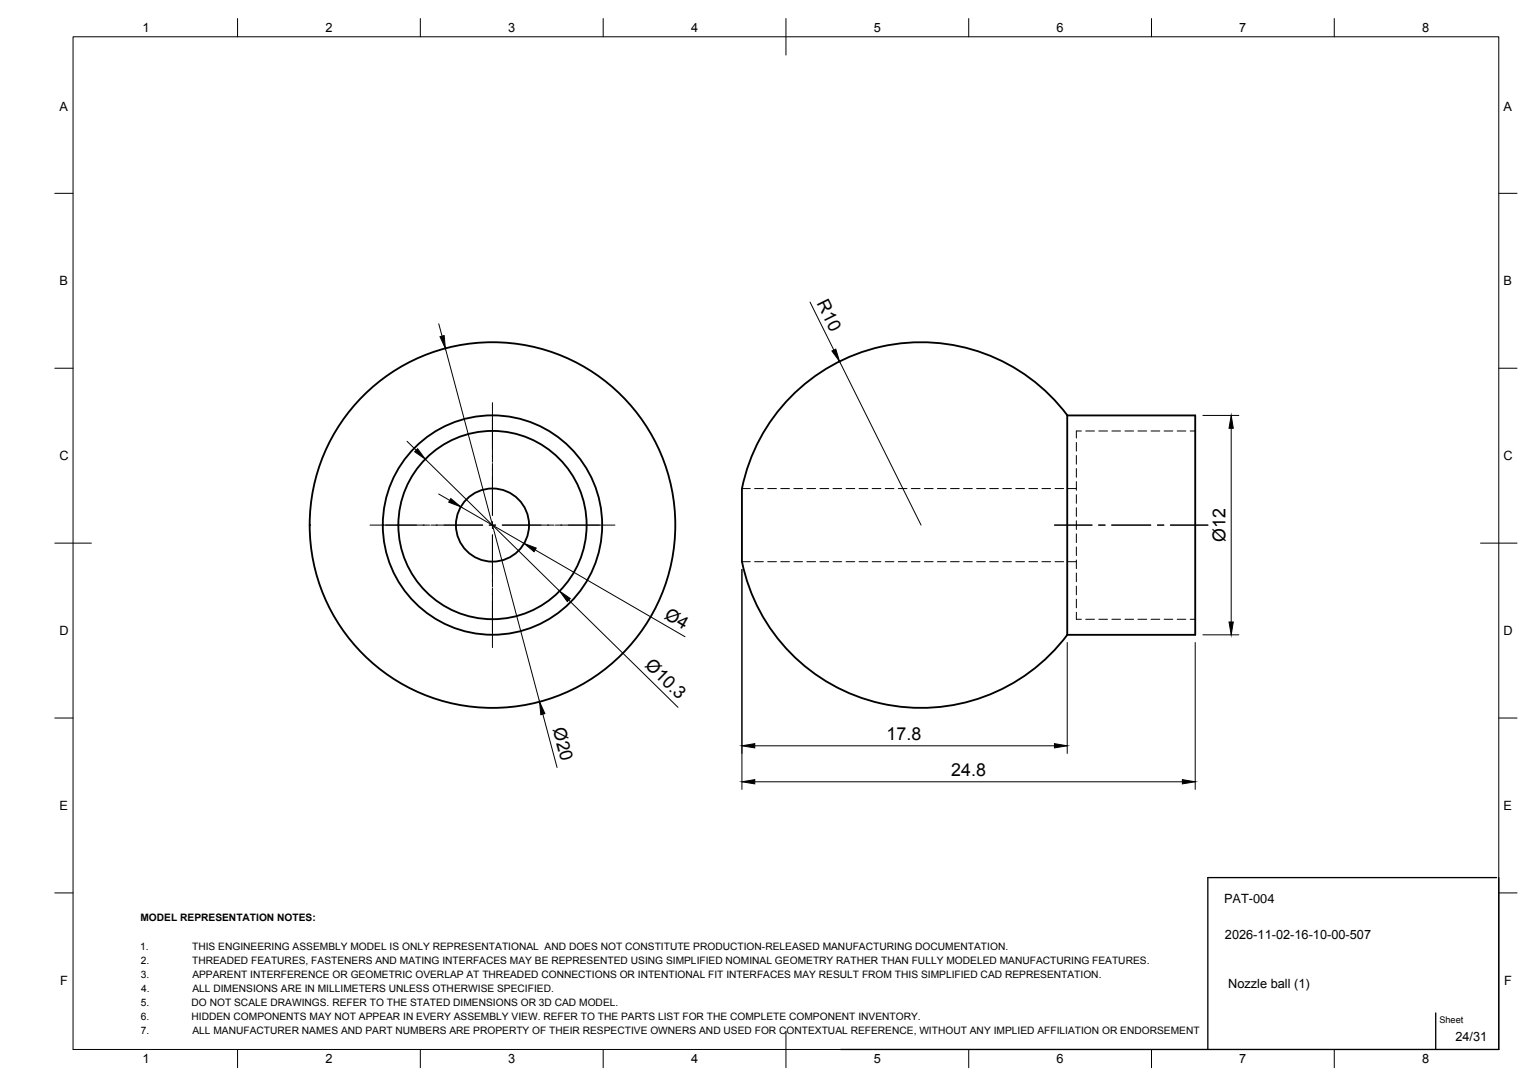
ISO-10303-21;
HEADER;
/* Generated by software containing ST-Developer
 * from STEP Tools, Inc. (www.steptools.com) 
 */

FILE_DESCRIPTION(
/* description */ ('Air blow-off nozzle station'),
/* implementation_level */ '2;1');

FILE_NAME(
/* name */ 'Nozzle ball (1).step',
/* time_stamp */ '2026-10-27T10:53:54-07:00',
/* author */ (''),
/* organization */ (''),
/* preprocessor_version */ 'ST-DEVELOPER v20.2',
/* originating_system */ 'Autodesk Translation Framework v15.17.0.0',
/* authorisation */ '');

FILE_SCHEMA (('AUTOMOTIVE_DESIGN { 1 0 10303 214 3 1 1 }'));
ENDSEC;

DATA;
#10=MECHANICAL_DESIGN_GEOMETRIC_PRESENTATION_REPRESENTATION('',(#254),#7897);
#169=SPHERICAL_SURFACE('',#4951,1.);
#204=SHAPE_REPRESENTATION_RELATIONSHIP('SRR','None',#8020,#229);
#229=ADVANCED_BREP_SHAPE_REPRESENTATION('',(#277),#7887);
#254=STYLED_ITEM('',(#8234),#277);
#277=MANIFOLD_SOLID_BREP('Body1',#4305);
#344=FACE_BOUND('',#1058,.T.);
#345=FACE_BOUND('',#1062,.T.);
#346=FACE_BOUND('',#1064,.T.);
#347=FACE_BOUND('',#1065,.T.);
#511=PLANE('',#4943);
#512=PLANE('',#4950);
#741=FACE_OUTER_BOUND('',#1056,.T.);
#742=FACE_OUTER_BOUND('',#1057,.T.);
#743=FACE_OUTER_BOUND('',#1059,.T.);
#744=FACE_OUTER_BOUND('',#1060,.T.);
#745=FACE_OUTER_BOUND('',#1061,.T.);
#746=FACE_OUTER_BOUND('',#1063,.T.);
#1056=EDGE_LOOP('',(#3775,#3776,#3777,#3778));
#1057=EDGE_LOOP('',(#3779));
#1058=EDGE_LOOP('',(#3780));
#1059=EDGE_LOOP('',(#3781,#3782,#3783,#3784));
#1060=EDGE_LOOP('',(#3785,#3786,#3787,#3788));
#1061=EDGE_LOOP('',(#3789));
#1062=EDGE_LOOP('',(#3790));
#1063=EDGE_LOOP('',(#3791,#3792));
#1064=EDGE_LOOP('',(#3793));
#1065=EDGE_LOOP('',(#3794));
#1450=LINE('',#7600,#1804);
#1451=LINE('',#7607,#1805);
#1452=LINE('',#7613,#1806);
#1804=VECTOR('',#6090,0.515);
#1805=VECTOR('',#6099,0.2);
#1806=VECTOR('',#6106,0.6);
#1957=CIRCLE('',#4941,0.515);
#1958=CIRCLE('',#4942,0.515);
#1959=CIRCLE('',#4944,0.2);
#1960=CIRCLE('',#4946,0.2);
#1961=CIRCLE('',#4948,0.6);
#1962=CIRCLE('',#4949,0.6);
#1963=CIRCLE('',#4952,1.);
#2302=VERTEX_POINT('',#7597);
#2303=VERTEX_POINT('',#7599);
#2304=VERTEX_POINT('',#7603);
#2305=VERTEX_POINT('',#7606);
#2306=VERTEX_POINT('',#7610);
#2307=VERTEX_POINT('',#7612);
#2308=VERTEX_POINT('',#7617);
#2309=VERTEX_POINT('',#7618);
#2805=EDGE_CURVE('',#2302,#2302,#1957,.T.);
#2806=EDGE_CURVE('',#2302,#2303,#1450,.T.);
#2807=EDGE_CURVE('',#2303,#2303,#1958,.T.);
#2808=EDGE_CURVE('',#2304,#2304,#1959,.T.);
#2809=EDGE_CURVE('',#2304,#2305,#1451,.T.);
#2810=EDGE_CURVE('',#2305,#2305,#1960,.T.);
#2811=EDGE_CURVE('',#2306,#2306,#1961,.T.);
#2812=EDGE_CURVE('',#2306,#2307,#1452,.T.);
#2813=EDGE_CURVE('',#2307,#2307,#1962,.T.);
#2814=EDGE_CURVE('',#2308,#2309,#1963,.T.);
#3775=ORIENTED_EDGE('',*,*,#2805,.F.);
#3776=ORIENTED_EDGE('',*,*,#2806,.T.);
#3777=ORIENTED_EDGE('',*,*,#2807,.T.);
#3778=ORIENTED_EDGE('',*,*,#2806,.F.);
#3779=ORIENTED_EDGE('',*,*,#2807,.F.);
#3780=ORIENTED_EDGE('',*,*,#2808,.F.);
#3781=ORIENTED_EDGE('',*,*,#2808,.T.);
#3782=ORIENTED_EDGE('',*,*,#2809,.T.);
#3783=ORIENTED_EDGE('',*,*,#2810,.F.);
#3784=ORIENTED_EDGE('',*,*,#2809,.F.);
#3785=ORIENTED_EDGE('',*,*,#2811,.F.);
#3786=ORIENTED_EDGE('',*,*,#2812,.T.);
#3787=ORIENTED_EDGE('',*,*,#2813,.T.);
#3788=ORIENTED_EDGE('',*,*,#2812,.F.);
#3789=ORIENTED_EDGE('',*,*,#2813,.F.);
#3790=ORIENTED_EDGE('',*,*,#2805,.T.);
#3791=ORIENTED_EDGE('',*,*,#2814,.T.);
#3792=ORIENTED_EDGE('',*,*,#2814,.F.);
#3793=ORIENTED_EDGE('',*,*,#2810,.T.);
#3794=ORIENTED_EDGE('',*,*,#2811,.T.);
#4006=CYLINDRICAL_SURFACE('',#4940,0.515);
#4007=CYLINDRICAL_SURFACE('',#4945,0.2);
#4008=CYLINDRICAL_SURFACE('',#4947,0.6);
#4231=ADVANCED_FACE('',(#741),#4006,.F.);
#4232=ADVANCED_FACE('',(#742,#344),#511,.F.);
#4233=ADVANCED_FACE('',(#743),#4007,.F.);
#4234=ADVANCED_FACE('',(#744),#4008,.T.);
#4235=ADVANCED_FACE('',(#745,#345),#512,.F.);
#4236=ADVANCED_FACE('',(#746,#346,#347),#169,.T.);
#4305=CLOSED_SHELL('',(#4231,#4232,#4233,#4234,#4235,#4236));
#4939=AXIS2_PLACEMENT_3D('',#7595,#6084,#6085);
#4940=AXIS2_PLACEMENT_3D('',#7596,#6086,#6087);
#4941=AXIS2_PLACEMENT_3D('',#7598,#6088,#6089);
#4942=AXIS2_PLACEMENT_3D('',#7601,#6091,#6092);
#4943=AXIS2_PLACEMENT_3D('',#7602,#6093,#6094);
#4944=AXIS2_PLACEMENT_3D('',#7604,#6095,#6096);
#4945=AXIS2_PLACEMENT_3D('',#7605,#6097,#6098);
#4946=AXIS2_PLACEMENT_3D('',#7608,#6100,#6101);
#4947=AXIS2_PLACEMENT_3D('',#7609,#6102,#6103);
#4948=AXIS2_PLACEMENT_3D('',#7611,#6104,#6105);
#4949=AXIS2_PLACEMENT_3D('',#7614,#6107,#6108);
#4950=AXIS2_PLACEMENT_3D('',#7615,#6109,#6110);
#4951=AXIS2_PLACEMENT_3D('',#7616,#6111,#6112);
#4952=AXIS2_PLACEMENT_3D('',#7619,#6113,#6114);
#6084=DIRECTION('axis',(0.,0.,1.));
#6085=DIRECTION('refdir',(1.,0.,0.));
#6086=DIRECTION('center_axis',(0.,1.,0.));
#6087=DIRECTION('ref_axis',(1.,0.,0.));
#6088=DIRECTION('center_axis',(0.,1.,0.));
#6089=DIRECTION('ref_axis',(1.,0.,0.));
#6090=DIRECTION('',(0.,1.,0.));
#6091=DIRECTION('center_axis',(0.,1.,0.));
#6092=DIRECTION('ref_axis',(1.,0.,0.));
#6093=DIRECTION('center_axis',(0.,1.,0.));
#6094=DIRECTION('ref_axis',(1.,0.,0.));
#6095=DIRECTION('center_axis',(0.,-1.,0.));
#6096=DIRECTION('ref_axis',(1.,0.,0.));
#6097=DIRECTION('center_axis',(0.,1.,0.));
#6098=DIRECTION('ref_axis',(1.,0.,0.));
#6099=DIRECTION('',(0.,1.,0.));
#6100=DIRECTION('center_axis',(0.,-1.,0.));
#6101=DIRECTION('ref_axis',(1.,-1.11022302462516E-15,0.));
#6102=DIRECTION('center_axis',(0.,1.,0.));
#6103=DIRECTION('ref_axis',(1.,0.,0.));
#6104=DIRECTION('center_axis',(0.,1.,0.));
#6105=DIRECTION('ref_axis',(1.,0.,0.));
#6106=DIRECTION('',(0.,-1.,0.));
#6107=DIRECTION('center_axis',(0.,1.,0.));
#6108=DIRECTION('ref_axis',(1.,0.,0.));
#6109=DIRECTION('center_axis',(0.,1.,0.));
#6110=DIRECTION('ref_axis',(1.,0.,0.));
#6111=DIRECTION('center_axis',(6.12323399573677E-17,0.,1.));
#6112=DIRECTION('ref_axis',(1.,0.,0.));
#6113=DIRECTION('center_axis',(0.,-1.,0.));
#6114=DIRECTION('ref_axis',(-1.,0.,0.));
#7595=CARTESIAN_POINT('',(0.,0.,0.));
#7596=CARTESIAN_POINT('Origin',(0.,-3.6,23.));
#7597=CARTESIAN_POINT('',(-0.515,-3.5,23.));
#7598=CARTESIAN_POINT('Origin',(0.,-3.5,23.));
#7599=CARTESIAN_POINT('',(-0.515,-2.85,23.));
#7600=CARTESIAN_POINT('',(-0.515,-3.6,23.));
#7601=CARTESIAN_POINT('Origin',(0.,-2.85,23.));
#7602=CARTESIAN_POINT('Origin',(0.,-2.85,23.));
#7603=CARTESIAN_POINT('',(-0.2,-2.85,23.));
#7604=CARTESIAN_POINT('Origin',(0.,-2.85,23.));
#7605=CARTESIAN_POINT('Origin',(0.,-3.6,23.));
#7606=CARTESIAN_POINT('',(-0.2,-1.02020410288673,23.));
#7607=CARTESIAN_POINT('',(-0.2,-3.6,23.));
#7608=CARTESIAN_POINT('Origin',(0.,-1.02020410288673,23.));
#7609=CARTESIAN_POINT('Origin',(0.,-3.5,23.));
#7610=CARTESIAN_POINT('',(-0.6,-2.8,23.));
#7611=CARTESIAN_POINT('Origin',(0.,-2.8,23.));
#7612=CARTESIAN_POINT('',(-0.6,-3.5,23.));
#7613=CARTESIAN_POINT('',(-0.6,-3.5,23.));
#7614=CARTESIAN_POINT('Origin',(0.,-3.5,23.));
#7615=CARTESIAN_POINT('Origin',(0.,-3.5,23.));
#7616=CARTESIAN_POINT('Origin',(0.,-2.,23.));
#7617=CARTESIAN_POINT('',(-6.12323399573677E-17,-2.,24.));
#7618=CARTESIAN_POINT('',(-6.12323399573677E-17,-2.,22.));
#7619=CARTESIAN_POINT('Origin',(0.,-2.,23.));
#7855=UNCERTAINTY_MEASURE_WITH_UNIT(LENGTH_MEASURE(0.001),#7898,
'DISTANCE_ACCURACY_VALUE',
'Maximum model space distance between geometric entities at asserted c
onnectivities');
#7865=UNCERTAINTY_MEASURE_WITH_UNIT(LENGTH_MEASURE(0.001),#7898,
'DISTANCE_ACCURACY_VALUE',
'Maximum model space distance between geometric entities at asserted c
onnectivities');
#7887=(
GEOMETRIC_REPRESENTATION_CONTEXT(3)
GLOBAL_UNCERTAINTY_ASSIGNED_CONTEXT((#7855))
GLOBAL_UNIT_ASSIGNED_CONTEXT((#7898,#7900,#7901))
REPRESENTATION_CONTEXT('','3D')
);
#7897=(
GEOMETRIC_REPRESENTATION_CONTEXT(3)
GLOBAL_UNCERTAINTY_ASSIGNED_CONTEXT((#7865))
GLOBAL_UNIT_ASSIGNED_CONTEXT((#7898,#7900,#7901))
REPRESENTATION_CONTEXT('','3D')
);
#7898=(
LENGTH_UNIT()
NAMED_UNIT(*)
SI_UNIT(.CENTI.,.METRE.)
);
#7900=(
NAMED_UNIT(*)
PLANE_ANGLE_UNIT()
SI_UNIT($,.RADIAN.)
);
#7901=(
NAMED_UNIT(*)
SI_UNIT($,.STERADIAN.)
SOLID_ANGLE_UNIT()
);
#7923=SHAPE_DEFINITION_REPRESENTATION(#7971,#8020);
#7971=PRODUCT_DEFINITION_SHAPE('',$,#8052);
#8020=SHAPE_REPRESENTATION('',(#4939),#7887);
#8030=PRODUCT_DEFINITION_CONTEXT('part definition',#8125,'design');
#8052=PRODUCT_DEFINITION('Nozzle ball (1)','Nozzle ball (1)',#8083,#8030);
#8083=PRODUCT_DEFINITION_FORMATION('',$,#8148);
#8125=APPLICATION_CONTEXT(
'Core Data for Automotive Mechanical Design Process');
#8126=PRODUCT_CONTEXT('part definition',#8125,'mechanical');
#8148=PRODUCT('Nozzle ball (1)','Nozzle ball (1)','Nozzle ball (1)',(#8126));
#8228=COLOUR_RGB('Off White',0.89,0.88,0.83);
#8229=FILL_AREA_STYLE_COLOUR('',#8228);
#8230=FILL_AREA_STYLE('',(#8229));
#8231=SURFACE_STYLE_FILL_AREA(#8230);
#8232=SURFACE_SIDE_STYLE('',(#8231));
#8233=SURFACE_STYLE_USAGE(.BOTH.,#8232);
#8234=PRESENTATION_STYLE_ASSIGNMENT((#8233));
ENDSEC;
END-ISO-10303-21;
